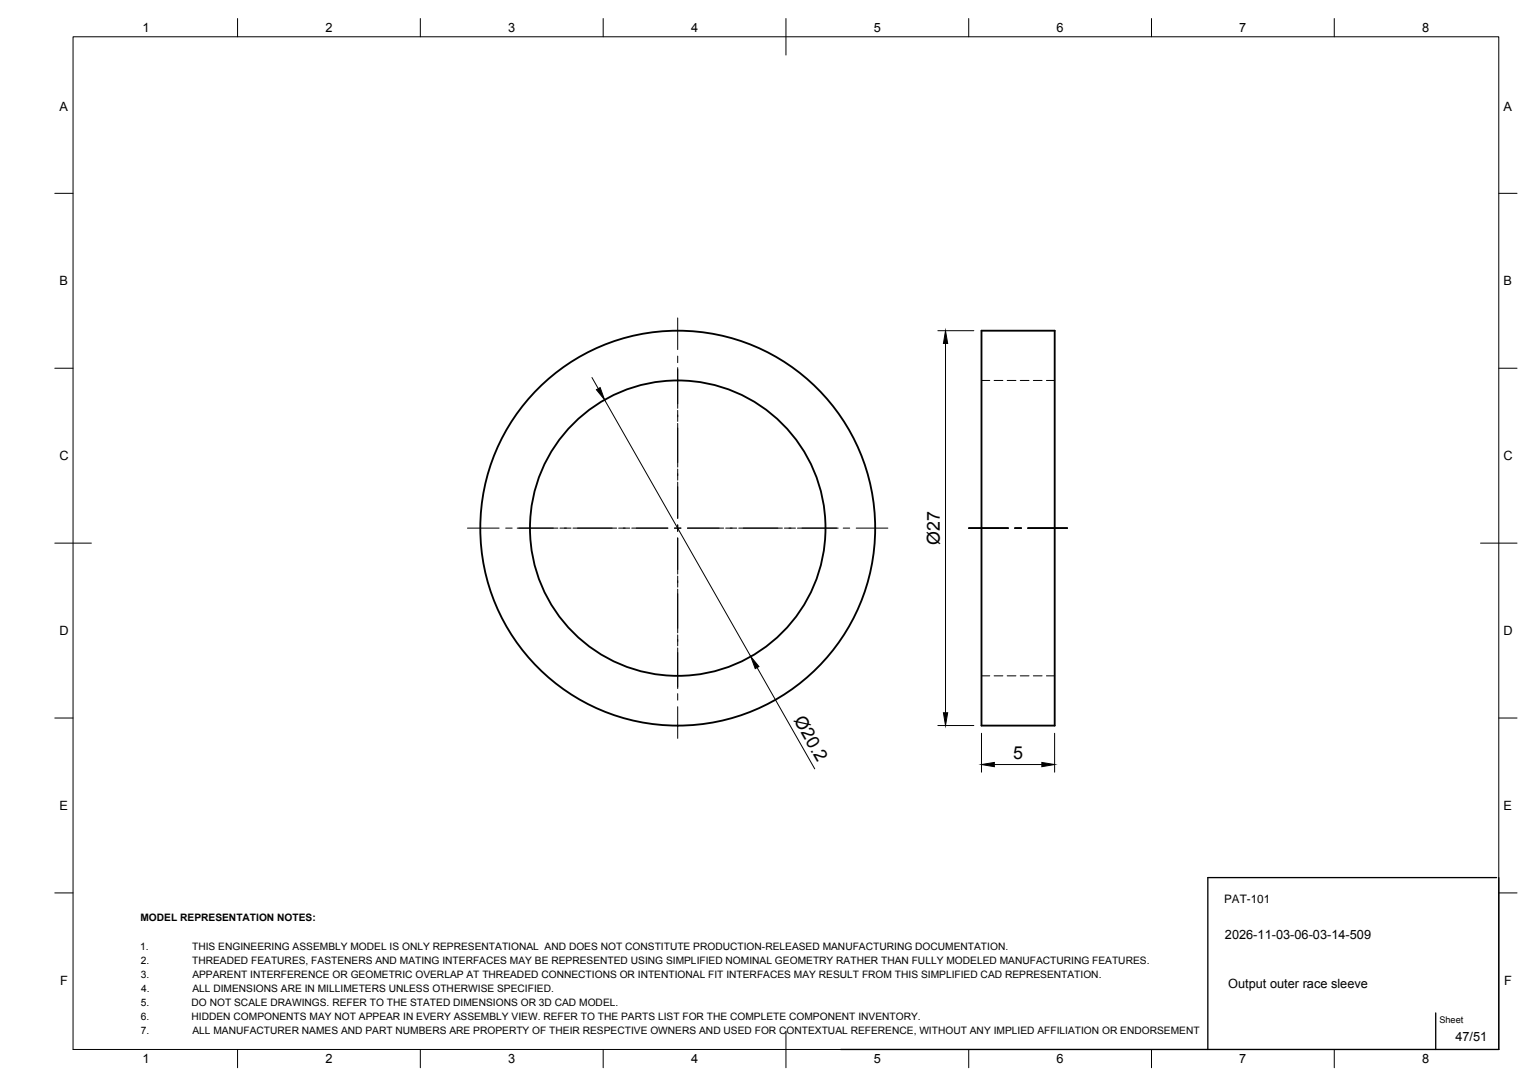
ISO-10303-21;
HEADER;
/* Generated by software containing ST-Developer
 * from STEP Tools, Inc. (www.steptools.com) 
 */

FILE_DESCRIPTION(
/* description */ ('Spur gear reduction stage 2-1 on bearing plates'),
/* implementation_level */ '2;1');

FILE_NAME(
/* name */ 'Output outer race sleeve.step',
/* time_stamp */ '2026-10-28T03:22:07-07:00',
/* author */ (''),
/* organization */ (''),
/* preprocessor_version */ 'ST-DEVELOPER v20.2',
/* originating_system */ 'Autodesk Translation Framework v15.17.0.0',
/* authorisation */ '');

FILE_SCHEMA (('AUTOMOTIVE_DESIGN { 1 0 10303 214 3 1 1 }'));
ENDSEC;

DATA;
#10=MECHANICAL_DESIGN_GEOMETRIC_PRESENTATION_REPRESENTATION('',(#999),#53909);
#898=SHAPE_REPRESENTATION_RELATIONSHIP('SRR','None',#54129,#941);
#941=ADVANCED_BREP_SHAPE_REPRESENTATION('',(#1054),#53903);
#999=STYLED_ITEM('',(#54397),#1054);
#1054=MANIFOLD_SOLID_BREP('Body1',#11326);
#1226=FACE_BOUND('',#2763,.T.);
#1227=FACE_BOUND('',#2765,.T.);
#1430=PLANE('',#12730);
#1431=PLANE('',#12731);
#1946=FACE_OUTER_BOUND('',#2760,.T.);
#1947=FACE_OUTER_BOUND('',#2761,.T.);
#1948=FACE_OUTER_BOUND('',#2762,.T.);
#1949=FACE_OUTER_BOUND('',#2764,.T.);
#2760=EDGE_LOOP('',(#9276,#9277,#9278,#9279));
#2761=EDGE_LOOP('',(#9280,#9281,#9282,#9283));
#2762=EDGE_LOOP('',(#9284));
#2763=EDGE_LOOP('',(#9285));
#2764=EDGE_LOOP('',(#9286));
#2765=EDGE_LOOP('',(#9287));
#3393=LINE('',#30006,#4034);
#3394=LINE('',#30012,#4035);
#4034=VECTOR('',#15238,1.01);
#4035=VECTOR('',#15245,1.35);
#4681=CIRCLE('',#12725,1.01);
#4682=CIRCLE('',#12726,1.01);
#4683=CIRCLE('',#12728,1.35);
#4684=CIRCLE('',#12729,1.35);
#5437=VERTEX_POINT('',#30003);
#5438=VERTEX_POINT('',#30005);
#5439=VERTEX_POINT('',#30009);
#5440=VERTEX_POINT('',#30011);
#6780=EDGE_CURVE('',#5437,#5437,#4681,.T.);
#6781=EDGE_CURVE('',#5437,#5438,#3393,.T.);
#6782=EDGE_CURVE('',#5438,#5438,#4682,.T.);
#6783=EDGE_CURVE('',#5439,#5439,#4683,.T.);
#6784=EDGE_CURVE('',#5439,#5440,#3394,.T.);
#6785=EDGE_CURVE('',#5440,#5440,#4684,.T.);
#9276=ORIENTED_EDGE('',*,*,#6780,.F.);
#9277=ORIENTED_EDGE('',*,*,#6781,.T.);
#9278=ORIENTED_EDGE('',*,*,#6782,.T.);
#9279=ORIENTED_EDGE('',*,*,#6781,.F.);
#9280=ORIENTED_EDGE('',*,*,#6783,.F.);
#9281=ORIENTED_EDGE('',*,*,#6784,.T.);
#9282=ORIENTED_EDGE('',*,*,#6785,.T.);
#9283=ORIENTED_EDGE('',*,*,#6784,.F.);
#9284=ORIENTED_EDGE('',*,*,#6783,.T.);
#9285=ORIENTED_EDGE('',*,*,#6780,.T.);
#9286=ORIENTED_EDGE('',*,*,#6785,.F.);
#9287=ORIENTED_EDGE('',*,*,#6782,.F.);
#10573=CYLINDRICAL_SURFACE('',#12724,1.01);
#10574=CYLINDRICAL_SURFACE('',#12727,1.35);
#11066=ADVANCED_FACE('',(#1946),#10573,.F.);
#11067=ADVANCED_FACE('',(#1947),#10574,.T.);
#11068=ADVANCED_FACE('',(#1948,#1226),#1430,.T.);
#11069=ADVANCED_FACE('',(#1949,#1227),#1431,.F.);
#11326=CLOSED_SHELL('',(#11066,#11067,#11068,#11069));
#12723=AXIS2_PLACEMENT_3D('',#30001,#15232,#15233);
#12724=AXIS2_PLACEMENT_3D('',#30002,#15234,#15235);
#12725=AXIS2_PLACEMENT_3D('',#30004,#15236,#15237);
#12726=AXIS2_PLACEMENT_3D('',#30007,#15239,#15240);
#12727=AXIS2_PLACEMENT_3D('',#30008,#15241,#15242);
#12728=AXIS2_PLACEMENT_3D('',#30010,#15243,#15244);
#12729=AXIS2_PLACEMENT_3D('',#30013,#15246,#15247);
#12730=AXIS2_PLACEMENT_3D('',#30014,#15248,#15249);
#12731=AXIS2_PLACEMENT_3D('',#30015,#15250,#15251);
#15232=DIRECTION('axis',(0.,0.,1.));
#15233=DIRECTION('refdir',(1.,0.,0.));
#15234=DIRECTION('center_axis',(0.,1.,0.));
#15235=DIRECTION('ref_axis',(1.,0.,0.));
#15236=DIRECTION('center_axis',(0.,-1.,0.));
#15237=DIRECTION('ref_axis',(1.,0.,0.));
#15238=DIRECTION('',(0.,-1.,0.));
#15239=DIRECTION('center_axis',(0.,-1.,0.));
#15240=DIRECTION('ref_axis',(1.,0.,0.));
#15241=DIRECTION('center_axis',(0.,1.,0.));
#15242=DIRECTION('ref_axis',(1.,0.,0.));
#15243=DIRECTION('center_axis',(0.,1.,0.));
#15244=DIRECTION('ref_axis',(1.,0.,0.));
#15245=DIRECTION('',(0.,-1.,0.));
#15246=DIRECTION('center_axis',(0.,1.,0.));
#15247=DIRECTION('ref_axis',(1.,0.,0.));
#15248=DIRECTION('center_axis',(0.,1.,0.));
#15249=DIRECTION('ref_axis',(1.,0.,0.));
#15250=DIRECTION('center_axis',(0.,1.,0.));
#15251=DIRECTION('ref_axis',(1.,0.,0.));
#30001=CARTESIAN_POINT('',(0.,0.,0.));
#30002=CARTESIAN_POINT('Origin',(0.,-4.7,0.));
#30003=CARTESIAN_POINT('',(-1.01,-4.2,1.23689326713883E-16));
#30004=CARTESIAN_POINT('Origin',(0.,-4.2,0.));
#30005=CARTESIAN_POINT('',(-1.01,-4.7,1.23689326713883E-16));
#30006=CARTESIAN_POINT('',(-1.01,-4.7,1.23689326713883E-16));
#30007=CARTESIAN_POINT('Origin',(0.,-4.7,0.));
#30008=CARTESIAN_POINT('Origin',(0.,-4.7,0.));
#30009=CARTESIAN_POINT('',(-1.35,-4.2,1.65327317884893E-16));
#30010=CARTESIAN_POINT('Origin',(0.,-4.2,0.));
#30011=CARTESIAN_POINT('',(-1.35,-4.7,1.65327317884893E-16));
#30012=CARTESIAN_POINT('',(-1.35,-4.7,1.65327317884893E-16));
#30013=CARTESIAN_POINT('Origin',(0.,-4.7,0.));
#30014=CARTESIAN_POINT('Origin',(0.,-4.2,0.));
#30015=CARTESIAN_POINT('Origin',(0.,-4.7,0.));
#53853=UNCERTAINTY_MEASURE_WITH_UNIT(LENGTH_MEASURE(0.001),#53910,
'DISTANCE_ACCURACY_VALUE',
'Maximum model space distance between geometric entities at asserted c
onnectivities');
#53859=UNCERTAINTY_MEASURE_WITH_UNIT(LENGTH_MEASURE(0.001),#53910,
'DISTANCE_ACCURACY_VALUE',
'Maximum model space distance between geometric entities at asserted c
onnectivities');
#53903=(
GEOMETRIC_REPRESENTATION_CONTEXT(3)
GLOBAL_UNCERTAINTY_ASSIGNED_CONTEXT((#53853))
GLOBAL_UNIT_ASSIGNED_CONTEXT((#53910,#53912,#53913))
REPRESENTATION_CONTEXT('','3D')
);
#53909=(
GEOMETRIC_REPRESENTATION_CONTEXT(3)
GLOBAL_UNCERTAINTY_ASSIGNED_CONTEXT((#53859))
GLOBAL_UNIT_ASSIGNED_CONTEXT((#53910,#53912,#53913))
REPRESENTATION_CONTEXT('','3D')
);
#53910=(
LENGTH_UNIT()
NAMED_UNIT(*)
SI_UNIT(.CENTI.,.METRE.)
);
#53912=(
NAMED_UNIT(*)
PLANE_ANGLE_UNIT()
SI_UNIT($,.RADIAN.)
);
#53913=(
NAMED_UNIT(*)
SI_UNIT($,.STERADIAN.)
SOLID_ANGLE_UNIT()
);
#53957=SHAPE_DEFINITION_REPRESENTATION(#54055,#54129);
#54055=PRODUCT_DEFINITION_SHAPE('',$,#54179);
#54129=SHAPE_REPRESENTATION('',(#12723),#53903);
#54135=PRODUCT_DEFINITION_CONTEXT('part definition',#54284,'design');
#54179=PRODUCT_DEFINITION('Output outer race sleeve',
'Output outer race sleeve',#54228,#54135);
#54228=PRODUCT_DEFINITION_FORMATION('',$,#54329);
#54284=APPLICATION_CONTEXT(
'Core Data for Automotive Mechanical Design Process');
#54285=PRODUCT_CONTEXT('part definition',#54284,'mechanical');
#54329=PRODUCT('Output outer race sleeve','Output outer race sleeve',
'Output outer race sleeve',(#54285));
#54391=COLOUR_RGB('Grey',0.48,0.52,0.57);
#54392=FILL_AREA_STYLE_COLOUR('',#54391);
#54393=FILL_AREA_STYLE('',(#54392));
#54394=SURFACE_STYLE_FILL_AREA(#54393);
#54395=SURFACE_SIDE_STYLE('',(#54394));
#54396=SURFACE_STYLE_USAGE(.BOTH.,#54395);
#54397=PRESENTATION_STYLE_ASSIGNMENT((#54396));
ENDSEC;
END-ISO-10303-21;
